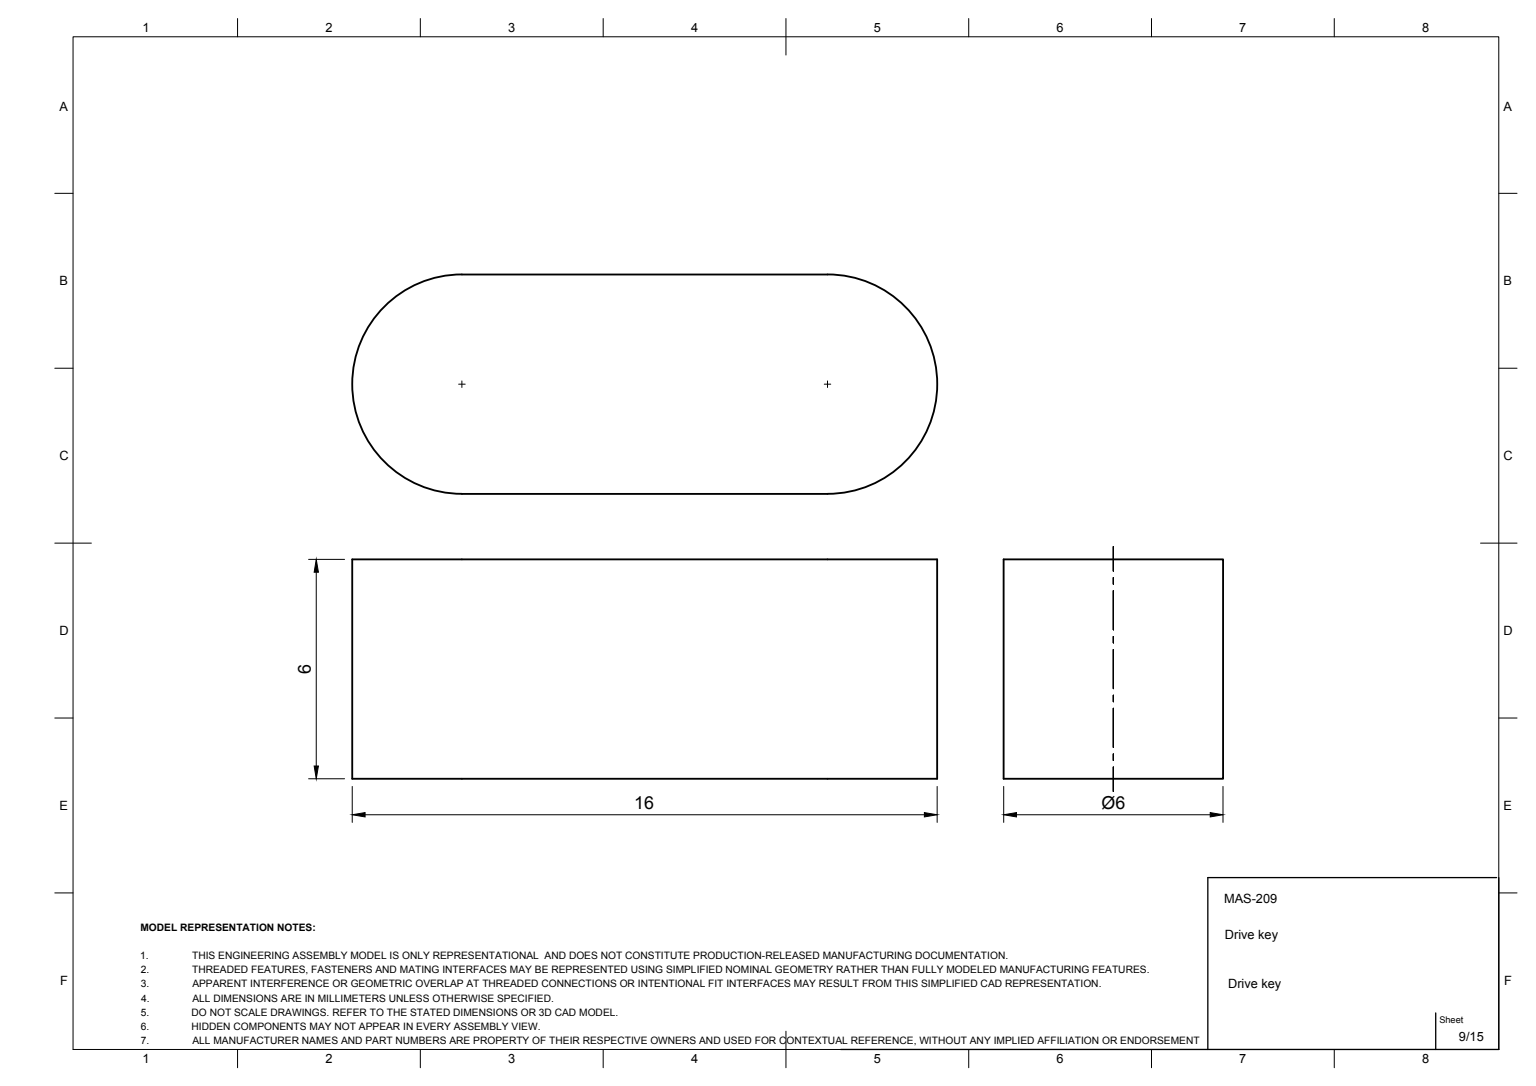
ISO-10303-21;
HEADER;
/* Generated by software containing ST-Developer
 * from STEP Tools, Inc. (www.steptools.com) 
 */

FILE_DESCRIPTION(
/* description */ ('Independent bearing-supported roller-ramp one-way clutch. Six logarit
hmic ramps with plain solid rollers, sprung guided plungers, native Co
il variants, removable shared keepers, rounded parallel key, shaft wit
h complete retaining lips, bronze journal/thrust support and bolted co
vers. Native rotor, roller planar/spin and plunger joints permit manua
l geometric engaged/released inspection. Automatic frictional torque s
witching/contact dynamics are not simulated; no capacity, hardness, fi
t, lubrication, speed, force or life rating. External input driver/cou
pling/anchors outside assembly.'),
/* implementation_level */ '2;1');

FILE_NAME(
/* name */ 'Drive key.step',
/* time_stamp */ '2026-11-08T07:04:38-08:00',
/* author */ (''),
/* organization */ (''),
/* preprocessor_version */ 'ST-DEVELOPER v20.2',
/* originating_system */ 'Autodesk Translation Framework v15.17.0.0',
/* authorisation */ '');

FILE_SCHEMA (('AUTOMOTIVE_DESIGN { 1 0 10303 214 3 1 1 }'));
ENDSEC;

DATA;
#10=MECHANICAL_DESIGN_GEOMETRIC_PRESENTATION_REPRESENTATION('',(#303),#99526);
#271=SHAPE_REPRESENTATION_RELATIONSHIP('SRR','None',#99628,#287);
#287=ADVANCED_BREP_SHAPE_REPRESENTATION('',(#319),#99513);
#303=STYLED_ITEM('',(#99717),#319);
#319=MANIFOLD_SOLID_BREP('Body1',#18273);
#561=PLANE('',#19479);
#562=PLANE('',#19483);
#563=PLANE('',#19487);
#564=PLANE('',#19488);
#1515=FACE_OUTER_BOUND('',#2574,.T.);
#1516=FACE_OUTER_BOUND('',#2575,.T.);
#1517=FACE_OUTER_BOUND('',#2576,.T.);
#1518=FACE_OUTER_BOUND('',#2577,.T.);
#1519=FACE_OUTER_BOUND('',#2578,.T.);
#1520=FACE_OUTER_BOUND('',#2579,.T.);
#2574=EDGE_LOOP('',(#15822,#15823,#15824,#15825));
#2575=EDGE_LOOP('',(#15826,#15827,#15828,#15829));
#2576=EDGE_LOOP('',(#15830,#15831,#15832,#15833));
#2577=EDGE_LOOP('',(#15834,#15835,#15836,#15837));
#2578=EDGE_LOOP('',(#15838,#15839,#15840,#15841));
#2579=EDGE_LOOP('',(#15842,#15843,#15844,#15845));
#3016=CIRCLE('',#19481,3.);
#3017=CIRCLE('',#19482,3.);
#3018=CIRCLE('',#19485,3.);
#3019=CIRCLE('',#19486,3.);
#5391=LINE('',#94634,#6295);
#5392=LINE('',#94636,#6296);
#5393=LINE('',#94638,#6297);
#5394=LINE('',#94639,#6298);
#5395=LINE('',#94645,#6299);
#5396=LINE('',#94648,#6300);
#5397=LINE('',#94650,#6301);
#5398=LINE('',#94651,#6302);
#6295=VECTOR('',#22594,10.);
#6296=VECTOR('',#22595,10.);
#6297=VECTOR('',#22596,10.);
#6298=VECTOR('',#22597,10.);
#6299=VECTOR('',#22604,10.);
#6300=VECTOR('',#22607,10.);
#6301=VECTOR('',#22608,10.);
#6302=VECTOR('',#22609,10.);
#8027=VERTEX_POINT('',#94632);
#8028=VERTEX_POINT('',#94633);
#8029=VERTEX_POINT('',#94635);
#8030=VERTEX_POINT('',#94637);
#8031=VERTEX_POINT('',#94641);
#8032=VERTEX_POINT('',#94643);
#8033=VERTEX_POINT('',#94647);
#8034=VERTEX_POINT('',#94649);
#10663=EDGE_CURVE('',#8027,#8028,#5391,.T.);
#10664=EDGE_CURVE('',#8027,#8029,#5392,.T.);
#10665=EDGE_CURVE('',#8030,#8029,#5393,.T.);
#10666=EDGE_CURVE('',#8028,#8030,#5394,.T.);
#10667=EDGE_CURVE('',#8031,#8028,#3016,.T.);
#10668=EDGE_CURVE('',#8032,#8030,#3017,.T.);
#10669=EDGE_CURVE('',#8031,#8032,#5395,.T.);
#10670=EDGE_CURVE('',#8031,#8033,#5396,.T.);
#10671=EDGE_CURVE('',#8034,#8032,#5397,.T.);
#10672=EDGE_CURVE('',#8033,#8034,#5398,.T.);
#10673=EDGE_CURVE('',#8027,#8033,#3018,.T.);
#10674=EDGE_CURVE('',#8029,#8034,#3019,.T.);
#15822=ORIENTED_EDGE('',*,*,#10663,.F.);
#15823=ORIENTED_EDGE('',*,*,#10664,.T.);
#15824=ORIENTED_EDGE('',*,*,#10665,.F.);
#15825=ORIENTED_EDGE('',*,*,#10666,.F.);
#15826=ORIENTED_EDGE('',*,*,#10667,.T.);
#15827=ORIENTED_EDGE('',*,*,#10666,.T.);
#15828=ORIENTED_EDGE('',*,*,#10668,.F.);
#15829=ORIENTED_EDGE('',*,*,#10669,.F.);
#15830=ORIENTED_EDGE('',*,*,#10670,.F.);
#15831=ORIENTED_EDGE('',*,*,#10669,.T.);
#15832=ORIENTED_EDGE('',*,*,#10671,.F.);
#15833=ORIENTED_EDGE('',*,*,#10672,.F.);
#15834=ORIENTED_EDGE('',*,*,#10673,.T.);
#15835=ORIENTED_EDGE('',*,*,#10672,.T.);
#15836=ORIENTED_EDGE('',*,*,#10674,.F.);
#15837=ORIENTED_EDGE('',*,*,#10664,.F.);
#15838=ORIENTED_EDGE('',*,*,#10674,.T.);
#15839=ORIENTED_EDGE('',*,*,#10671,.T.);
#15840=ORIENTED_EDGE('',*,*,#10668,.T.);
#15841=ORIENTED_EDGE('',*,*,#10665,.T.);
#15842=ORIENTED_EDGE('',*,*,#10673,.F.);
#15843=ORIENTED_EDGE('',*,*,#10663,.T.);
#15844=ORIENTED_EDGE('',*,*,#10667,.F.);
#15845=ORIENTED_EDGE('',*,*,#10670,.T.);
#17183=CYLINDRICAL_SURFACE('',#19480,3.);
#17184=CYLINDRICAL_SURFACE('',#19484,3.);
#18113=ADVANCED_FACE('',(#1515),#561,.T.);
#18114=ADVANCED_FACE('',(#1516),#17183,.T.);
#18115=ADVANCED_FACE('',(#1517),#562,.T.);
#18116=ADVANCED_FACE('',(#1518),#17184,.T.);
#18117=ADVANCED_FACE('',(#1519),#563,.T.);
#18118=ADVANCED_FACE('',(#1520),#564,.F.);
#18273=CLOSED_SHELL('',(#18113,#18114,#18115,#18116,#18117,#18118));
#19478=AXIS2_PLACEMENT_3D('',#94630,#22590,#22591);
#19479=AXIS2_PLACEMENT_3D('',#94631,#22592,#22593);
#19480=AXIS2_PLACEMENT_3D('',#94640,#22598,#22599);
#19481=AXIS2_PLACEMENT_3D('',#94642,#22600,#22601);
#19482=AXIS2_PLACEMENT_3D('',#94644,#22602,#22603);
#19483=AXIS2_PLACEMENT_3D('',#94646,#22605,#22606);
#19484=AXIS2_PLACEMENT_3D('',#94652,#22610,#22611);
#19485=AXIS2_PLACEMENT_3D('',#94653,#22612,#22613);
#19486=AXIS2_PLACEMENT_3D('',#94654,#22614,#22615);
#19487=AXIS2_PLACEMENT_3D('',#94655,#22616,#22617);
#19488=AXIS2_PLACEMENT_3D('',#94656,#22618,#22619);
#22590=DIRECTION('axis',(0.,0.,1.));
#22591=DIRECTION('refdir',(1.,0.,0.));
#22592=DIRECTION('center_axis',(0.,1.,0.));
#22593=DIRECTION('ref_axis',(0.,0.,1.));
#22594=DIRECTION('',(0.,0.,-1.));
#22595=DIRECTION('',(1.,0.,0.));
#22596=DIRECTION('',(0.,0.,1.));
#22597=DIRECTION('',(1.,0.,0.));
#22598=DIRECTION('center_axis',(1.,0.,0.));
#22599=DIRECTION('ref_axis',(0.,-1.,0.));
#22600=DIRECTION('center_axis',(1.,0.,0.));
#22601=DIRECTION('ref_axis',(0.,-1.,0.));
#22602=DIRECTION('center_axis',(1.,0.,0.));
#22603=DIRECTION('ref_axis',(0.,-1.,0.));
#22604=DIRECTION('',(1.,0.,0.));
#22605=DIRECTION('center_axis',(0.,-1.,0.));
#22606=DIRECTION('ref_axis',(0.,0.,-1.));
#22607=DIRECTION('',(0.,0.,1.));
#22608=DIRECTION('',(0.,0.,-1.));
#22609=DIRECTION('',(1.,0.,0.));
#22610=DIRECTION('center_axis',(1.,0.,0.));
#22611=DIRECTION('ref_axis',(0.,1.,0.));
#22612=DIRECTION('center_axis',(1.,0.,0.));
#22613=DIRECTION('ref_axis',(0.,1.,0.));
#22614=DIRECTION('center_axis',(1.,0.,0.));
#22615=DIRECTION('ref_axis',(0.,1.,0.));
#22616=DIRECTION('center_axis',(1.,0.,0.));
#22617=DIRECTION('ref_axis',(0.,0.,-1.));
#22618=DIRECTION('center_axis',(1.,0.,0.));
#22619=DIRECTION('ref_axis',(0.,0.,-1.));
#94630=CARTESIAN_POINT('',(0.,0.,0.));
#94631=CARTESIAN_POINT('Origin',(0.,3.,5.));
#94632=CARTESIAN_POINT('',(0.,3.,15.));
#94633=CARTESIAN_POINT('',(0.,3.,5.));
#94634=CARTESIAN_POINT('',(0.,3.,15.));
#94635=CARTESIAN_POINT('',(6.,3.,15.));
#94636=CARTESIAN_POINT('',(0.,3.,15.));
#94637=CARTESIAN_POINT('',(6.,3.,5.));
#94638=CARTESIAN_POINT('',(6.,3.,15.));
#94639=CARTESIAN_POINT('',(0.,3.,5.));
#94640=CARTESIAN_POINT('Origin',(0.,0.,5.));
#94641=CARTESIAN_POINT('',(0.,-3.,5.));
#94642=CARTESIAN_POINT('Origin',(0.,0.,5.));
#94643=CARTESIAN_POINT('',(6.,-3.,5.));
#94644=CARTESIAN_POINT('Origin',(6.,0.,5.));
#94645=CARTESIAN_POINT('',(0.,-3.,5.));
#94646=CARTESIAN_POINT('Origin',(0.,-3.,15.));
#94647=CARTESIAN_POINT('',(0.,-3.,15.));
#94648=CARTESIAN_POINT('',(0.,-3.,5.));
#94649=CARTESIAN_POINT('',(6.,-3.,15.));
#94650=CARTESIAN_POINT('',(6.,-3.,5.));
#94651=CARTESIAN_POINT('',(0.,-3.,15.));
#94652=CARTESIAN_POINT('Origin',(0.,0.,15.));
#94653=CARTESIAN_POINT('Origin',(0.,0.,15.));
#94654=CARTESIAN_POINT('Origin',(6.,0.,15.));
#94655=CARTESIAN_POINT('Origin',(6.,0.,10.));
#94656=CARTESIAN_POINT('Origin',(0.,0.,10.));
#99495=UNCERTAINTY_MEASURE_WITH_UNIT(LENGTH_MEASURE(0.01),#99527,
'DISTANCE_ACCURACY_VALUE',
'Maximum model space distance between geometric entities at asserted c
onnectivities');
#99508=UNCERTAINTY_MEASURE_WITH_UNIT(LENGTH_MEASURE(0.01),#99527,
'DISTANCE_ACCURACY_VALUE',
'Maximum model space distance between geometric entities at asserted c
onnectivities');
#99513=(
GEOMETRIC_REPRESENTATION_CONTEXT(3)
GLOBAL_UNCERTAINTY_ASSIGNED_CONTEXT((#99495))
GLOBAL_UNIT_ASSIGNED_CONTEXT((#99527,#99529,#99530))
REPRESENTATION_CONTEXT('','3D')
);
#99526=(
GEOMETRIC_REPRESENTATION_CONTEXT(3)
GLOBAL_UNCERTAINTY_ASSIGNED_CONTEXT((#99508))
GLOBAL_UNIT_ASSIGNED_CONTEXT((#99527,#99529,#99530))
REPRESENTATION_CONTEXT('','3D')
);
#99527=(
LENGTH_UNIT()
NAMED_UNIT(*)
SI_UNIT(.MILLI.,.METRE.)
);
#99529=(
NAMED_UNIT(*)
PLANE_ANGLE_UNIT()
SI_UNIT($,.RADIAN.)
);
#99530=(
NAMED_UNIT(*)
SI_UNIT($,.STERADIAN.)
SOLID_ANGLE_UNIT()
);
#99535=SHAPE_DEFINITION_REPRESENTATION(#99552,#99628);
#99552=PRODUCT_DEFINITION_SHAPE('',$,#99646);
#99628=SHAPE_REPRESENTATION('',(#19478),#99513);
#99641=PRODUCT_DEFINITION_CONTEXT('part definition',#99694,'design');
#99646=PRODUCT_DEFINITION('Drive key','Drive key',#99663,#99641);
#99663=PRODUCT_DEFINITION_FORMATION('',$,#99700);
#99694=APPLICATION_CONTEXT(
'Core Data for Automotive Mechanical Design Process');
#99695=PRODUCT_CONTEXT('part definition',#99694,'mechanical');
#99700=PRODUCT('Drive key','Drive key',$,(#99695));
#99717=PRESENTATION_STYLE_ASSIGNMENT((#99730));
#99730=SURFACE_STYLE_USAGE(.BOTH.,#99743);
#99743=SURFACE_SIDE_STYLE('',(#99756));
#99756=SURFACE_STYLE_FILL_AREA(#99769);
#99769=FILL_AREA_STYLE('Light gray',(#99782));
#99782=FILL_AREA_STYLE_COLOUR('Light gray',#99795);
#99795=COLOUR_RGB('Light gray',0.725490196078431,0.752941176470588,0.792156862745098);
ENDSEC;
END-ISO-10303-21;
